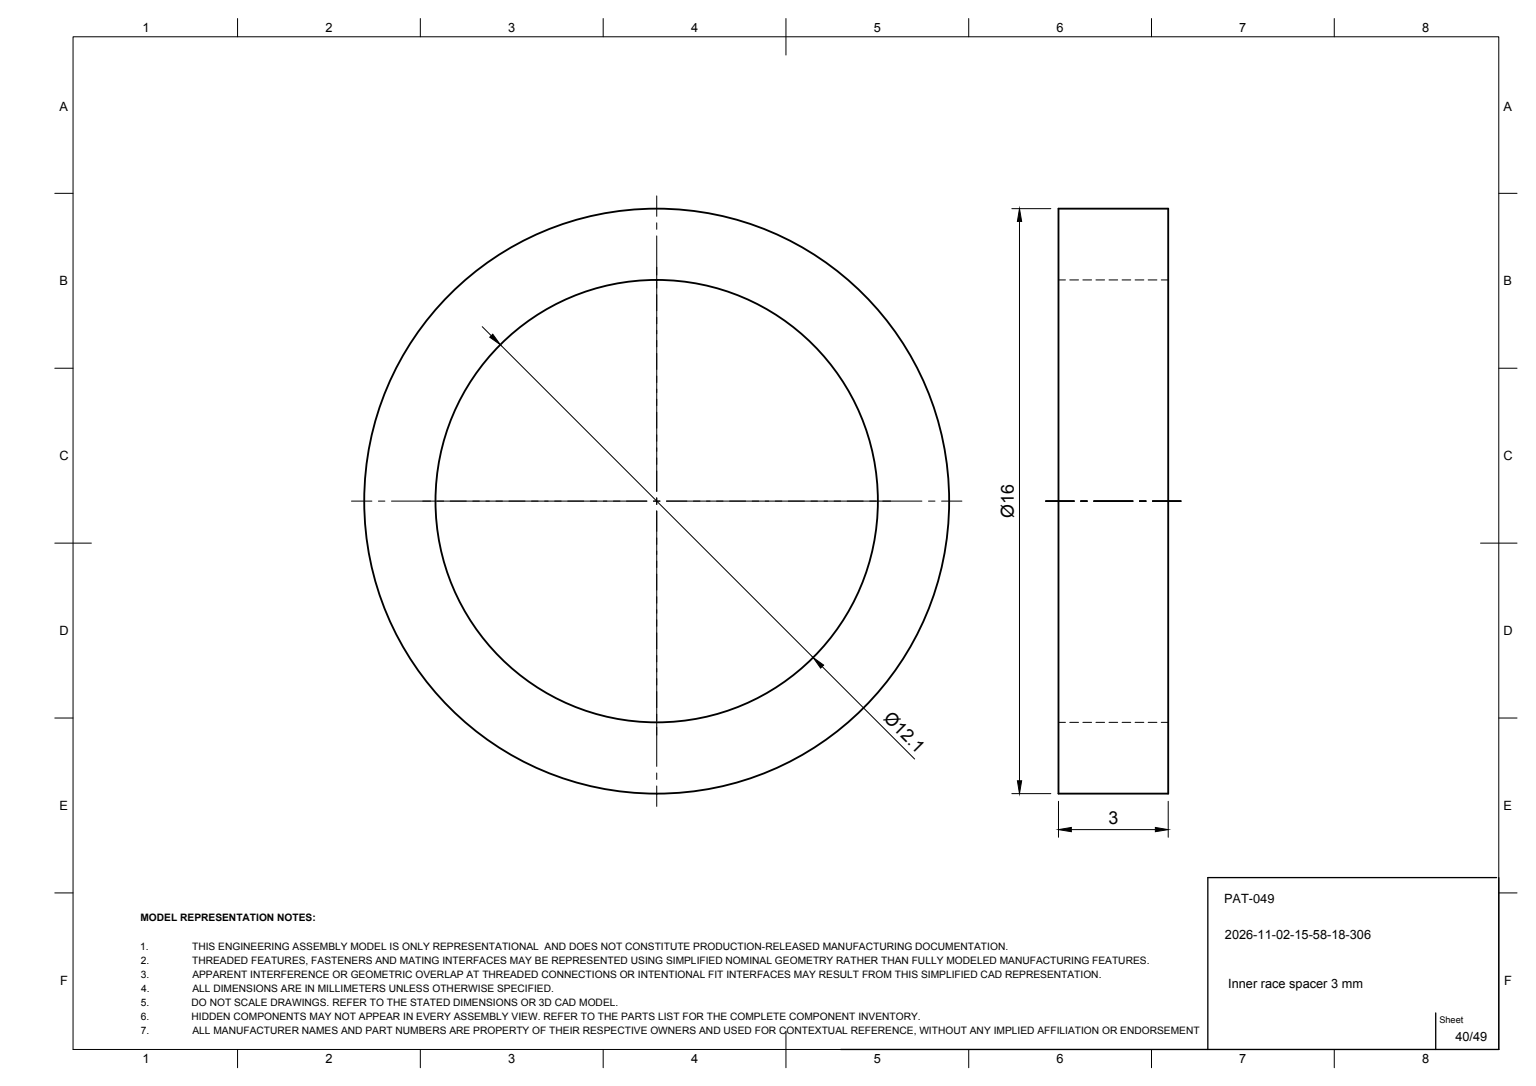
ISO-10303-21;
HEADER;
/* Generated by software containing ST-Developer
 * from STEP Tools, Inc. (www.steptools.com) 
 */

FILE_DESCRIPTION(
/* description */ ('Hand drill press frame (manual)'),
/* implementation_level */ '2;1');

FILE_NAME(
/* name */ 'Inner race spacer 3 mm.step',
/* time_stamp */ '2026-10-28T03:25:28-07:00',
/* author */ (''),
/* organization */ (''),
/* preprocessor_version */ 'ST-DEVELOPER v20.2',
/* originating_system */ 'Autodesk Translation Framework v15.17.0.0',
/* authorisation */ '');

FILE_SCHEMA (('AUTOMOTIVE_DESIGN { 1 0 10303 214 3 1 1 }'));
ENDSEC;

DATA;
#10=MECHANICAL_DESIGN_GEOMETRIC_PRESENTATION_REPRESENTATION('',(#658),#33299);
#561=SHAPE_REPRESENTATION_RELATIONSHIP('SRR','None',#33523,#606);
#606=ADVANCED_BREP_SHAPE_REPRESENTATION('',(#709),#33285);
#658=STYLED_ITEM('',(#33814),#709);
#709=MANIFOLD_SOLID_BREP('Body1',#12677);
#863=FACE_BOUND('',#2688,.T.);
#864=FACE_BOUND('',#2690,.T.);
#1256=PLANE('',#14058);
#1257=PLANE('',#14059);
#1853=FACE_OUTER_BOUND('',#2685,.T.);
#1854=FACE_OUTER_BOUND('',#2686,.T.);
#1855=FACE_OUTER_BOUND('',#2687,.T.);
#1856=FACE_OUTER_BOUND('',#2689,.T.);
#2685=EDGE_LOOP('',(#10955,#10956,#10957,#10958));
#2686=EDGE_LOOP('',(#10959,#10960,#10961,#10962));
#2687=EDGE_LOOP('',(#10963));
#2688=EDGE_LOOP('',(#10964));
#2689=EDGE_LOOP('',(#10965));
#2690=EDGE_LOOP('',(#10966));
#3812=LINE('',#21174,#4977);
#3813=LINE('',#21180,#4978);
#4977=VECTOR('',#17027,0.605);
#4978=VECTOR('',#17034,0.8);
#5515=CIRCLE('',#14053,0.605);
#5516=CIRCLE('',#14054,0.605);
#5517=CIRCLE('',#14056,0.8);
#5518=CIRCLE('',#14057,0.8);
#6465=VERTEX_POINT('',#21171);
#6466=VERTEX_POINT('',#21173);
#6467=VERTEX_POINT('',#21177);
#6468=VERTEX_POINT('',#21179);
#8006=EDGE_CURVE('',#6465,#6465,#5515,.T.);
#8007=EDGE_CURVE('',#6465,#6466,#3812,.T.);
#8008=EDGE_CURVE('',#6466,#6466,#5516,.T.);
#8009=EDGE_CURVE('',#6467,#6467,#5517,.T.);
#8010=EDGE_CURVE('',#6467,#6468,#3813,.T.);
#8011=EDGE_CURVE('',#6468,#6468,#5518,.T.);
#10955=ORIENTED_EDGE('',*,*,#8006,.F.);
#10956=ORIENTED_EDGE('',*,*,#8007,.T.);
#10957=ORIENTED_EDGE('',*,*,#8008,.T.);
#10958=ORIENTED_EDGE('',*,*,#8007,.F.);
#10959=ORIENTED_EDGE('',*,*,#8009,.F.);
#10960=ORIENTED_EDGE('',*,*,#8010,.T.);
#10961=ORIENTED_EDGE('',*,*,#8011,.T.);
#10962=ORIENTED_EDGE('',*,*,#8010,.F.);
#10963=ORIENTED_EDGE('',*,*,#8009,.T.);
#10964=ORIENTED_EDGE('',*,*,#8006,.T.);
#10965=ORIENTED_EDGE('',*,*,#8011,.F.);
#10966=ORIENTED_EDGE('',*,*,#8008,.F.);
#11904=CYLINDRICAL_SURFACE('',#14052,0.605);
#11905=CYLINDRICAL_SURFACE('',#14055,0.8);
#12462=ADVANCED_FACE('',(#1853),#11904,.F.);
#12463=ADVANCED_FACE('',(#1854),#11905,.T.);
#12464=ADVANCED_FACE('',(#1855,#863),#1256,.T.);
#12465=ADVANCED_FACE('',(#1856,#864),#1257,.F.);
#12677=CLOSED_SHELL('',(#12462,#12463,#12464,#12465));
#14051=AXIS2_PLACEMENT_3D('',#21169,#17021,#17022);
#14052=AXIS2_PLACEMENT_3D('',#21170,#17023,#17024);
#14053=AXIS2_PLACEMENT_3D('',#21172,#17025,#17026);
#14054=AXIS2_PLACEMENT_3D('',#21175,#17028,#17029);
#14055=AXIS2_PLACEMENT_3D('',#21176,#17030,#17031);
#14056=AXIS2_PLACEMENT_3D('',#21178,#17032,#17033);
#14057=AXIS2_PLACEMENT_3D('',#21181,#17035,#17036);
#14058=AXIS2_PLACEMENT_3D('',#21182,#17037,#17038);
#14059=AXIS2_PLACEMENT_3D('',#21183,#17039,#17040);
#17021=DIRECTION('axis',(0.,0.,1.));
#17022=DIRECTION('refdir',(1.,0.,0.));
#17023=DIRECTION('center_axis',(0.,1.,0.));
#17024=DIRECTION('ref_axis',(1.,0.,0.));
#17025=DIRECTION('center_axis',(0.,-1.,0.));
#17026=DIRECTION('ref_axis',(1.,0.,0.));
#17027=DIRECTION('',(0.,-1.,0.));
#17028=DIRECTION('center_axis',(0.,-1.,0.));
#17029=DIRECTION('ref_axis',(1.,0.,0.));
#17030=DIRECTION('center_axis',(0.,1.,0.));
#17031=DIRECTION('ref_axis',(1.,0.,0.));
#17032=DIRECTION('center_axis',(0.,1.,0.));
#17033=DIRECTION('ref_axis',(1.,0.,0.));
#17034=DIRECTION('',(0.,-1.,0.));
#17035=DIRECTION('center_axis',(0.,1.,0.));
#17036=DIRECTION('ref_axis',(1.,0.,0.));
#17037=DIRECTION('center_axis',(0.,1.,0.));
#17038=DIRECTION('ref_axis',(1.,0.,0.));
#17039=DIRECTION('center_axis',(0.,1.,0.));
#17040=DIRECTION('ref_axis',(1.,0.,0.));
#21169=CARTESIAN_POINT('',(0.,0.,0.));
#21170=CARTESIAN_POINT('Origin',(-3.25,2.2,20.));
#21171=CARTESIAN_POINT('',(-3.855,2.5,20.));
#21172=CARTESIAN_POINT('Origin',(-3.25,2.5,20.));
#21173=CARTESIAN_POINT('',(-3.855,2.2,20.));
#21174=CARTESIAN_POINT('',(-3.855,2.2,20.));
#21175=CARTESIAN_POINT('Origin',(-3.25,2.2,20.));
#21176=CARTESIAN_POINT('Origin',(-3.25,2.2,20.));
#21177=CARTESIAN_POINT('',(-4.05,2.5,20.));
#21178=CARTESIAN_POINT('Origin',(-3.25,2.5,20.));
#21179=CARTESIAN_POINT('',(-4.05,2.2,20.));
#21180=CARTESIAN_POINT('',(-4.05,2.2,20.));
#21181=CARTESIAN_POINT('Origin',(-3.25,2.2,20.));
#21182=CARTESIAN_POINT('Origin',(-3.25,2.5,20.));
#21183=CARTESIAN_POINT('Origin',(-3.25,2.2,20.));
#33233=UNCERTAINTY_MEASURE_WITH_UNIT(LENGTH_MEASURE(0.001),#33300,
'DISTANCE_ACCURACY_VALUE',
'Maximum model space distance between geometric entities at asserted c
onnectivities');
#33247=UNCERTAINTY_MEASURE_WITH_UNIT(LENGTH_MEASURE(0.001),#33300,
'DISTANCE_ACCURACY_VALUE',
'Maximum model space distance between geometric entities at asserted c
onnectivities');
#33285=(
GEOMETRIC_REPRESENTATION_CONTEXT(3)
GLOBAL_UNCERTAINTY_ASSIGNED_CONTEXT((#33233))
GLOBAL_UNIT_ASSIGNED_CONTEXT((#33300,#33302,#33303))
REPRESENTATION_CONTEXT('','3D')
);
#33299=(
GEOMETRIC_REPRESENTATION_CONTEXT(3)
GLOBAL_UNCERTAINTY_ASSIGNED_CONTEXT((#33247))
GLOBAL_UNIT_ASSIGNED_CONTEXT((#33300,#33302,#33303))
REPRESENTATION_CONTEXT('','3D')
);
#33300=(
LENGTH_UNIT()
NAMED_UNIT(*)
SI_UNIT(.CENTI.,.METRE.)
);
#33302=(
NAMED_UNIT(*)
PLANE_ANGLE_UNIT()
SI_UNIT($,.RADIAN.)
);
#33303=(
NAMED_UNIT(*)
SI_UNIT($,.STERADIAN.)
SOLID_ANGLE_UNIT()
);
#33341=SHAPE_DEFINITION_REPRESENTATION(#33403,#33523);
#33403=PRODUCT_DEFINITION_SHAPE('',$,#33575);
#33523=SHAPE_REPRESENTATION('',(#14051),#33285);
#33537=PRODUCT_DEFINITION_CONTEXT('part definition',#33692,'design');
#33575=PRODUCT_DEFINITION('Inner race spacer 3 mm',
'Inner race spacer 3 mm',#33626,#33537);
#33626=PRODUCT_DEFINITION_FORMATION('',$,#33731);
#33692=APPLICATION_CONTEXT(
'Core Data for Automotive Mechanical Design Process');
#33693=PRODUCT_CONTEXT('part definition',#33692,'mechanical');
#33731=PRODUCT('Inner race spacer 3 mm','Inner race spacer 3 mm',
'Inner race spacer 3 mm',(#33693));
#33808=COLOUR_RGB('Grey',0.48,0.52,0.57);
#33809=FILL_AREA_STYLE_COLOUR('',#33808);
#33810=FILL_AREA_STYLE('',(#33809));
#33811=SURFACE_STYLE_FILL_AREA(#33810);
#33812=SURFACE_SIDE_STYLE('',(#33811));
#33813=SURFACE_STYLE_USAGE(.BOTH.,#33812);
#33814=PRESENTATION_STYLE_ASSIGNMENT((#33813));
ENDSEC;
END-ISO-10303-21;
